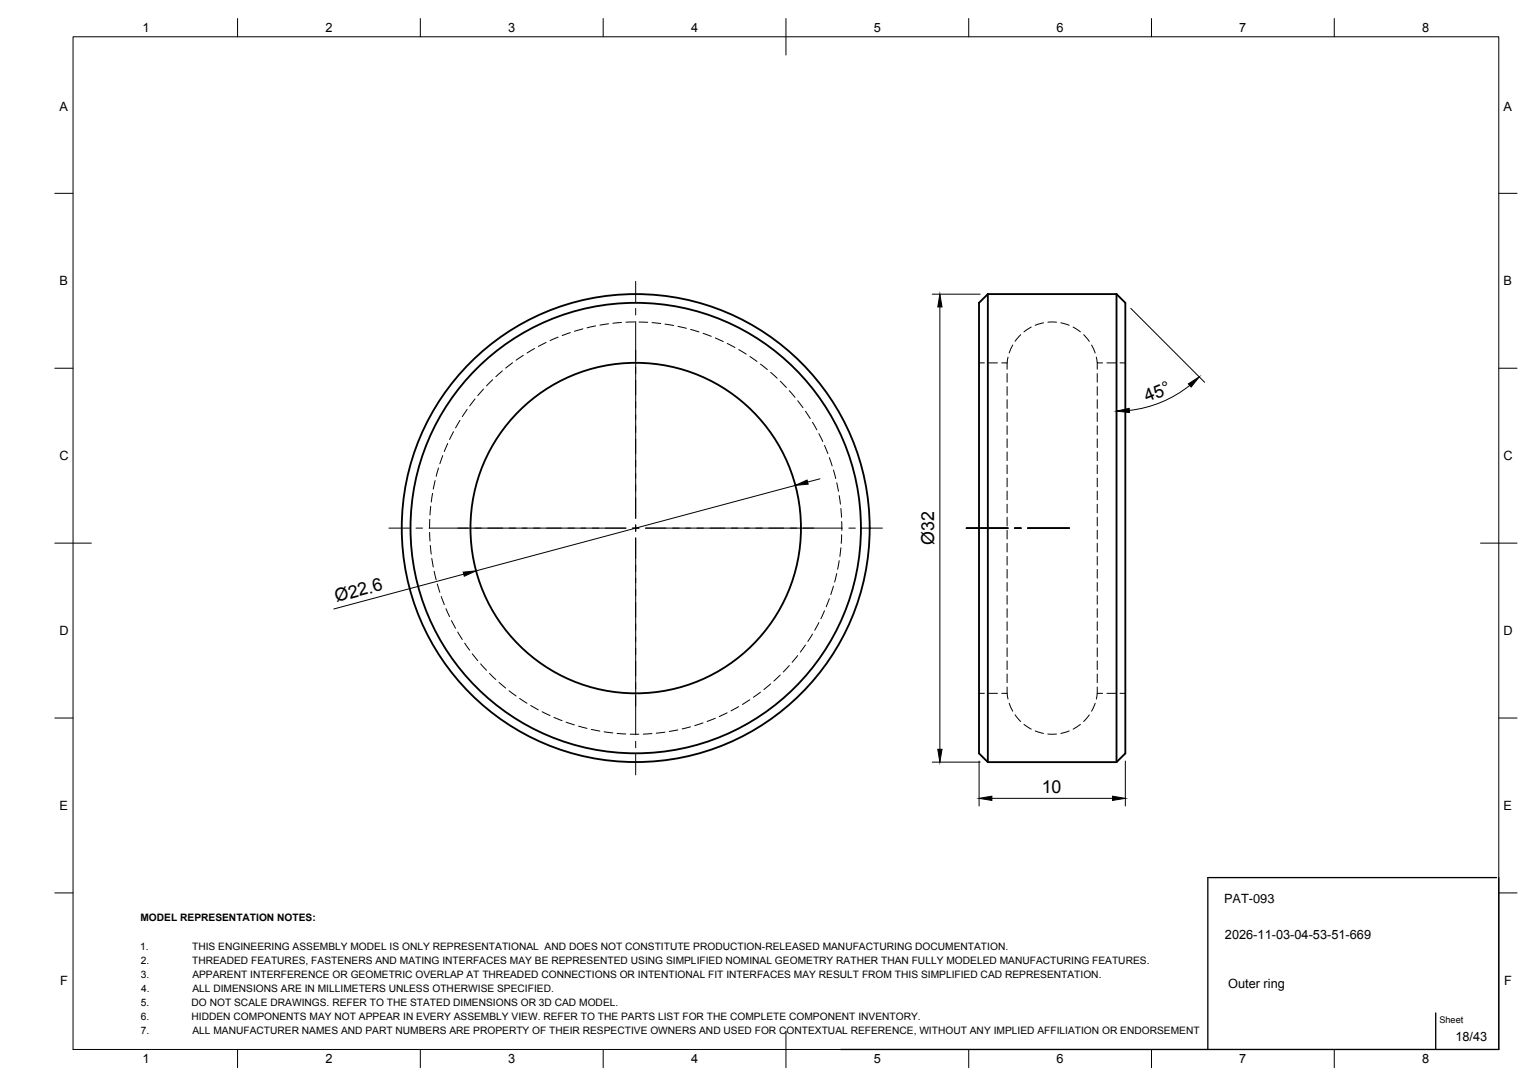
ISO-10303-21;
HEADER;
/* Generated by software containing ST-Developer
 * from STEP Tools, Inc. (www.steptools.com) 
 */

FILE_DESCRIPTION(
/* description */ ('Self-centering screw clamp'),
/* implementation_level */ '2;1');

FILE_NAME(
/* name */ 'Outer ring.step',
/* time_stamp */ '2026-10-28T03:25:31-07:00',
/* author */ (''),
/* organization */ (''),
/* preprocessor_version */ 'ST-DEVELOPER v20.2',
/* originating_system */ 'Autodesk Translation Framework v15.17.0.0',
/* authorisation */ '');

FILE_SCHEMA (('AUTOMOTIVE_DESIGN { 1 0 10303 214 3 1 1 }'));
ENDSEC;

DATA;
#10=MECHANICAL_DESIGN_GEOMETRIC_PRESENTATION_REPRESENTATION('',(#639),#16799);
#482=TOROIDAL_SURFACE('',#9976,1.1,0.309556);
#487=CONICAL_SURFACE('',#9987,1.57,0.785398163397449);
#488=CONICAL_SURFACE('',#9991,1.57,0.785398163397449);
#557=SHAPE_REPRESENTATION_RELATIONSHIP('SRR','None',#17031,#598);
#598=ADVANCED_BREP_SHAPE_REPRESENTATION('',(#687),#16769);
#639=STYLED_ITEM('',(#17326),#687);
#687=MANIFOLD_SOLID_BREP('Body1',#9090);
#844=FACE_BOUND('',#2095,.T.);
#845=FACE_BOUND('',#2100,.T.);
#1108=PLANE('',#9984);
#1109=PLANE('',#9993);
#1462=FACE_OUTER_BOUND('',#2092,.T.);
#1463=FACE_OUTER_BOUND('',#2093,.T.);
#1464=FACE_OUTER_BOUND('',#2094,.T.);
#1465=FACE_OUTER_BOUND('',#2096,.T.);
#1466=FACE_OUTER_BOUND('',#2097,.T.);
#1467=FACE_OUTER_BOUND('',#2098,.T.);
#1468=FACE_OUTER_BOUND('',#2099,.T.);
#1469=FACE_OUTER_BOUND('',#2101,.T.);
#2092=EDGE_LOOP('',(#7025,#7026,#7027,#7028,#7029,#7030));
#2093=EDGE_LOOP('',(#7031,#7032,#7033,#7034,#7035));
#2094=EDGE_LOOP('',(#7036));
#2095=EDGE_LOOP('',(#7037));
#2096=EDGE_LOOP('',(#7038,#7039,#7040,#7041));
#2097=EDGE_LOOP('',(#7042,#7043,#7044,#7045));
#2098=EDGE_LOOP('',(#7046,#7047,#7048,#7049));
#2099=EDGE_LOOP('',(#7050));
#2100=EDGE_LOOP('',(#7051));
#2101=EDGE_LOOP('',(#7052,#7053,#7054,#7055,#7056));
#2831=LINE('',#14731,#3404);
#2832=LINE('',#14740,#3405);
#2833=LINE('',#14744,#3406);
#2834=LINE('',#14748,#3407);
#2835=LINE('',#14751,#3408);
#3404=VECTOR('',#11820,1.129765);
#3405=VECTOR('',#11831,1.57);
#3406=VECTOR('',#11836,1.6);
#3407=VECTOR('',#11841,1.57);
#3408=VECTOR('',#11846,1.129765);
#3914=CIRCLE('',#9977,1.129765);
#3915=CIRCLE('',#9978,1.129765);
#3916=CIRCLE('',#9979,0.309556);
#3917=CIRCLE('',#9980,1.129765);
#3918=CIRCLE('',#9981,1.129765);
#3919=CIRCLE('',#9983,1.129765);
#3920=CIRCLE('',#9985,1.54);
#3921=CIRCLE('',#9986,1.129765);
#3922=CIRCLE('',#9988,1.6);
#3923=CIRCLE('',#9990,1.6);
#3924=CIRCLE('',#9992,1.54);
#4527=VERTEX_POINT('',#14719);
#4528=VERTEX_POINT('',#14720);
#4529=VERTEX_POINT('',#14723);
#4530=VERTEX_POINT('',#14725);
#4531=VERTEX_POINT('',#14729);
#4532=VERTEX_POINT('',#14733);
#4533=VERTEX_POINT('',#14735);
#4534=VERTEX_POINT('',#14738);
#4535=VERTEX_POINT('',#14742);
#4536=VERTEX_POINT('',#14746);
#5437=EDGE_CURVE('',#4527,#4528,#3914,.T.);
#5438=EDGE_CURVE('',#4528,#4527,#3915,.T.);
#5439=EDGE_CURVE('',#4528,#4529,#3916,.T.);
#5440=EDGE_CURVE('',#4530,#4529,#3917,.T.);
#5441=EDGE_CURVE('',#4529,#4530,#3918,.T.);
#5442=EDGE_CURVE('',#4531,#4531,#3919,.T.);
#5443=EDGE_CURVE('',#4531,#4530,#2831,.T.);
#5444=EDGE_CURVE('',#4532,#4532,#3920,.T.);
#5445=EDGE_CURVE('',#4533,#4533,#3921,.T.);
#5446=EDGE_CURVE('',#4534,#4534,#3922,.T.);
#5447=EDGE_CURVE('',#4534,#4532,#2832,.T.);
#5448=EDGE_CURVE('',#4535,#4535,#3923,.T.);
#5449=EDGE_CURVE('',#4535,#4534,#2833,.T.);
#5450=EDGE_CURVE('',#4536,#4536,#3924,.T.);
#5451=EDGE_CURVE('',#4536,#4535,#2834,.T.);
#5452=EDGE_CURVE('',#4527,#4533,#2835,.T.);
#7025=ORIENTED_EDGE('',*,*,#5437,.F.);
#7026=ORIENTED_EDGE('',*,*,#5438,.F.);
#7027=ORIENTED_EDGE('',*,*,#5439,.T.);
#7028=ORIENTED_EDGE('',*,*,#5440,.F.);
#7029=ORIENTED_EDGE('',*,*,#5441,.F.);
#7030=ORIENTED_EDGE('',*,*,#5439,.F.);
#7031=ORIENTED_EDGE('',*,*,#5442,.T.);
#7032=ORIENTED_EDGE('',*,*,#5443,.T.);
#7033=ORIENTED_EDGE('',*,*,#5440,.T.);
#7034=ORIENTED_EDGE('',*,*,#5441,.T.);
#7035=ORIENTED_EDGE('',*,*,#5443,.F.);
#7036=ORIENTED_EDGE('',*,*,#5444,.F.);
#7037=ORIENTED_EDGE('',*,*,#5445,.T.);
#7038=ORIENTED_EDGE('',*,*,#5446,.F.);
#7039=ORIENTED_EDGE('',*,*,#5447,.T.);
#7040=ORIENTED_EDGE('',*,*,#5444,.T.);
#7041=ORIENTED_EDGE('',*,*,#5447,.F.);
#7042=ORIENTED_EDGE('',*,*,#5448,.F.);
#7043=ORIENTED_EDGE('',*,*,#5449,.T.);
#7044=ORIENTED_EDGE('',*,*,#5446,.T.);
#7045=ORIENTED_EDGE('',*,*,#5449,.F.);
#7046=ORIENTED_EDGE('',*,*,#5450,.F.);
#7047=ORIENTED_EDGE('',*,*,#5451,.T.);
#7048=ORIENTED_EDGE('',*,*,#5448,.T.);
#7049=ORIENTED_EDGE('',*,*,#5451,.F.);
#7050=ORIENTED_EDGE('',*,*,#5450,.T.);
#7051=ORIENTED_EDGE('',*,*,#5442,.F.);
#7052=ORIENTED_EDGE('',*,*,#5437,.T.);
#7053=ORIENTED_EDGE('',*,*,#5438,.T.);
#7054=ORIENTED_EDGE('',*,*,#5452,.T.);
#7055=ORIENTED_EDGE('',*,*,#5445,.F.);
#7056=ORIENTED_EDGE('',*,*,#5452,.F.);
#8447=CYLINDRICAL_SURFACE('',#9982,1.129765);
#8448=CYLINDRICAL_SURFACE('',#9989,1.6);
#8449=CYLINDRICAL_SURFACE('',#9994,1.129765);
#8760=ADVANCED_FACE('',(#1462),#482,.F.);
#8761=ADVANCED_FACE('',(#1463),#8447,.F.);
#8762=ADVANCED_FACE('',(#1464,#844),#1108,.T.);
#8763=ADVANCED_FACE('',(#1465),#487,.T.);
#8764=ADVANCED_FACE('',(#1466),#8448,.T.);
#8765=ADVANCED_FACE('',(#1467),#488,.T.);
#8766=ADVANCED_FACE('',(#1468,#845),#1109,.T.);
#8767=ADVANCED_FACE('',(#1469),#8449,.F.);
#9090=CLOSED_SHELL('',(#8760,#8761,#8762,#8763,#8764,#8765,#8766,#8767));
#9975=AXIS2_PLACEMENT_3D('',#14717,#11802,#11803);
#9976=AXIS2_PLACEMENT_3D('',#14718,#11804,#11805);
#9977=AXIS2_PLACEMENT_3D('',#14721,#11806,#11807);
#9978=AXIS2_PLACEMENT_3D('',#14722,#11808,#11809);
#9979=AXIS2_PLACEMENT_3D('',#14724,#11810,#11811);
#9980=AXIS2_PLACEMENT_3D('',#14726,#11812,#11813);
#9981=AXIS2_PLACEMENT_3D('',#14727,#11814,#11815);
#9982=AXIS2_PLACEMENT_3D('',#14728,#11816,#11817);
#9983=AXIS2_PLACEMENT_3D('',#14730,#11818,#11819);
#9984=AXIS2_PLACEMENT_3D('',#14732,#11821,#11822);
#9985=AXIS2_PLACEMENT_3D('',#14734,#11823,#11824);
#9986=AXIS2_PLACEMENT_3D('',#14736,#11825,#11826);
#9987=AXIS2_PLACEMENT_3D('',#14737,#11827,#11828);
#9988=AXIS2_PLACEMENT_3D('',#14739,#11829,#11830);
#9989=AXIS2_PLACEMENT_3D('',#14741,#11832,#11833);
#9990=AXIS2_PLACEMENT_3D('',#14743,#11834,#11835);
#9991=AXIS2_PLACEMENT_3D('',#14745,#11837,#11838);
#9992=AXIS2_PLACEMENT_3D('',#14747,#11839,#11840);
#9993=AXIS2_PLACEMENT_3D('',#14749,#11842,#11843);
#9994=AXIS2_PLACEMENT_3D('',#14750,#11844,#11845);
#11802=DIRECTION('axis',(0.,0.,1.));
#11803=DIRECTION('refdir',(1.,0.,0.));
#11804=DIRECTION('center_axis',(0.,-1.,0.));
#11805=DIRECTION('ref_axis',(0.,0.,-1.));
#11806=DIRECTION('center_axis',(0.,-1.,0.));
#11807=DIRECTION('ref_axis',(1.,0.,0.));
#11808=DIRECTION('center_axis',(0.,-1.,0.));
#11809=DIRECTION('ref_axis',(1.,0.,0.));
#11810=DIRECTION('center_axis',(1.,0.,1.22464679914735E-16));
#11811=DIRECTION('ref_axis',(-1.22464679914735E-16,0.,1.));
#11812=DIRECTION('center_axis',(0.,1.,0.));
#11813=DIRECTION('ref_axis',(1.,0.,0.));
#11814=DIRECTION('center_axis',(0.,1.,0.));
#11815=DIRECTION('ref_axis',(1.,0.,0.));
#11816=DIRECTION('center_axis',(0.,-1.,0.));
#11817=DIRECTION('ref_axis',(1.,0.,0.));
#11818=DIRECTION('center_axis',(0.,-1.,0.));
#11819=DIRECTION('ref_axis',(1.,0.,0.));
#11820=DIRECTION('',(0.,1.,0.));
#11821=DIRECTION('center_axis',(0.,1.,0.));
#11822=DIRECTION('ref_axis',(0.,0.,1.));
#11823=DIRECTION('center_axis',(0.,-1.,0.));
#11824=DIRECTION('ref_axis',(1.,0.,0.));
#11825=DIRECTION('center_axis',(0.,-1.,0.));
#11826=DIRECTION('ref_axis',(1.,0.,0.));
#11827=DIRECTION('center_axis',(0.,-1.,0.));
#11828=DIRECTION('ref_axis',(1.,0.,0.));
#11829=DIRECTION('center_axis',(0.,-1.,0.));
#11830=DIRECTION('ref_axis',(1.,0.,0.));
#11831=DIRECTION('',(0.707106781186548,0.707106781186547,8.65956056235494E-17));
#11832=DIRECTION('center_axis',(0.,-1.,0.));
#11833=DIRECTION('ref_axis',(1.,0.,0.));
#11834=DIRECTION('center_axis',(0.,-1.,0.));
#11835=DIRECTION('ref_axis',(1.,0.,0.));
#11836=DIRECTION('',(0.,1.,0.));
#11837=DIRECTION('center_axis',(0.,1.,0.));
#11838=DIRECTION('ref_axis',(1.,0.,0.));
#11839=DIRECTION('center_axis',(0.,-1.,0.));
#11840=DIRECTION('ref_axis',(1.,0.,0.));
#11841=DIRECTION('',(-0.707106781186548,0.707106781186547,-8.65956056235494E-17));
#11842=DIRECTION('center_axis',(0.,-1.,0.));
#11843=DIRECTION('ref_axis',(0.,0.,-1.));
#11844=DIRECTION('center_axis',(0.,-1.,0.));
#11845=DIRECTION('ref_axis',(1.,0.,0.));
#11846=DIRECTION('',(0.,1.,0.));
#14717=CARTESIAN_POINT('',(0.,0.,0.));
#14718=CARTESIAN_POINT('Origin',(0.,0.,0.));
#14719=CARTESIAN_POINT('',(-1.129765,0.308121667383195,-1.38356309103871E-16));
#14720=CARTESIAN_POINT('',(-1.38356309103871E-16,0.308121667383195,1.129765));
#14721=CARTESIAN_POINT('Origin',(0.,0.308121667383195,0.));
#14722=CARTESIAN_POINT('Origin',(0.,0.308121667383195,0.));
#14723=CARTESIAN_POINT('',(-1.38356309103871E-16,-0.308121667383195,1.129765));
#14724=CARTESIAN_POINT('Origin',(-1.34711147906209E-16,0.,1.1));
#14725=CARTESIAN_POINT('',(-1.129765,-0.308121667383195,1.38356309103871E-16));
#14726=CARTESIAN_POINT('Origin',(0.,-0.308121667383195,0.));
#14727=CARTESIAN_POINT('Origin',(0.,-0.308121667383195,0.));
#14728=CARTESIAN_POINT('Origin',(0.,0.,0.));
#14729=CARTESIAN_POINT('',(-1.129765,-0.5,-1.38356309103871E-16));
#14730=CARTESIAN_POINT('Origin',(0.,-0.5,0.));
#14731=CARTESIAN_POINT('',(-1.129765,0.,-1.38356309103871E-16));
#14732=CARTESIAN_POINT('Origin',(1.54,0.5,0.));
#14733=CARTESIAN_POINT('',(-1.54,0.5,-1.88595607068692E-16));
#14734=CARTESIAN_POINT('Origin',(0.,0.5,0.));
#14735=CARTESIAN_POINT('',(-1.129765,0.5,-1.38356309103871E-16));
#14736=CARTESIAN_POINT('Origin',(0.,0.5,0.));
#14737=CARTESIAN_POINT('Origin',(0.,0.47,0.));
#14738=CARTESIAN_POINT('',(-1.6,0.44,-1.95943487863577E-16));
#14739=CARTESIAN_POINT('Origin',(0.,0.44,0.));
#14740=CARTESIAN_POINT('',(-1.57,0.47,-1.92269547466134E-16));
#14741=CARTESIAN_POINT('Origin',(0.,0.,0.));
#14742=CARTESIAN_POINT('',(-1.6,-0.44,-1.95943487863577E-16));
#14743=CARTESIAN_POINT('Origin',(0.,-0.44,0.));
#14744=CARTESIAN_POINT('',(-1.6,0.,-1.95943487863577E-16));
#14745=CARTESIAN_POINT('Origin',(0.,-0.47,0.));
#14746=CARTESIAN_POINT('',(-1.54,-0.5,-1.88595607068692E-16));
#14747=CARTESIAN_POINT('Origin',(0.,-0.5,0.));
#14748=CARTESIAN_POINT('',(-1.57,-0.47,-1.92269547466134E-16));
#14749=CARTESIAN_POINT('Origin',(1.129765,-0.5,0.));
#14750=CARTESIAN_POINT('Origin',(0.,0.,0.));
#14751=CARTESIAN_POINT('',(-1.129765,0.,-1.38356309103871E-16));
#16720=UNCERTAINTY_MEASURE_WITH_UNIT(LENGTH_MEASURE(0.001),#16800,
'DISTANCE_ACCURACY_VALUE',
'Maximum model space distance between geometric entities at asserted c
onnectivities');
#16750=UNCERTAINTY_MEASURE_WITH_UNIT(LENGTH_MEASURE(0.001),#16800,
'DISTANCE_ACCURACY_VALUE',
'Maximum model space distance between geometric entities at asserted c
onnectivities');
#16769=(
GEOMETRIC_REPRESENTATION_CONTEXT(3)
GLOBAL_UNCERTAINTY_ASSIGNED_CONTEXT((#16720))
GLOBAL_UNIT_ASSIGNED_CONTEXT((#16800,#16802,#16803))
REPRESENTATION_CONTEXT('','3D')
);
#16799=(
GEOMETRIC_REPRESENTATION_CONTEXT(3)
GLOBAL_UNCERTAINTY_ASSIGNED_CONTEXT((#16750))
GLOBAL_UNIT_ASSIGNED_CONTEXT((#16800,#16802,#16803))
REPRESENTATION_CONTEXT('','3D')
);
#16800=(
LENGTH_UNIT()
NAMED_UNIT(*)
SI_UNIT(.CENTI.,.METRE.)
);
#16802=(
NAMED_UNIT(*)
PLANE_ANGLE_UNIT()
SI_UNIT($,.RADIAN.)
);
#16803=(
NAMED_UNIT(*)
SI_UNIT($,.STERADIAN.)
SOLID_ANGLE_UNIT()
);
#16822=SHAPE_DEFINITION_REPRESENTATION(#16870,#17031);
#16870=PRODUCT_DEFINITION_SHAPE('',$,#17080);
#17031=SHAPE_REPRESENTATION('',(#9975),#16769);
#17061=PRODUCT_DEFINITION_CONTEXT('part definition',#17207,'design');
#17080=PRODUCT_DEFINITION('Outer ring','Outer ring',#17128,#17061);
#17128=PRODUCT_DEFINITION_FORMATION('',$,#17227);
#17207=APPLICATION_CONTEXT(
'Core Data for Automotive Mechanical Design Process');
#17208=PRODUCT_CONTEXT('part definition',#17207,'mechanical');
#17227=PRODUCT('Outer ring','Outer ring','Outer ring',(#17208));
#17320=COLOUR_RGB('Grey',0.48,0.52,0.57);
#17321=FILL_AREA_STYLE_COLOUR('',#17320);
#17322=FILL_AREA_STYLE('',(#17321));
#17323=SURFACE_STYLE_FILL_AREA(#17322);
#17324=SURFACE_SIDE_STYLE('',(#17323));
#17325=SURFACE_STYLE_USAGE(.BOTH.,#17324);
#17326=PRESENTATION_STYLE_ASSIGNMENT((#17325));
ENDSEC;
END-ISO-10303-21;
